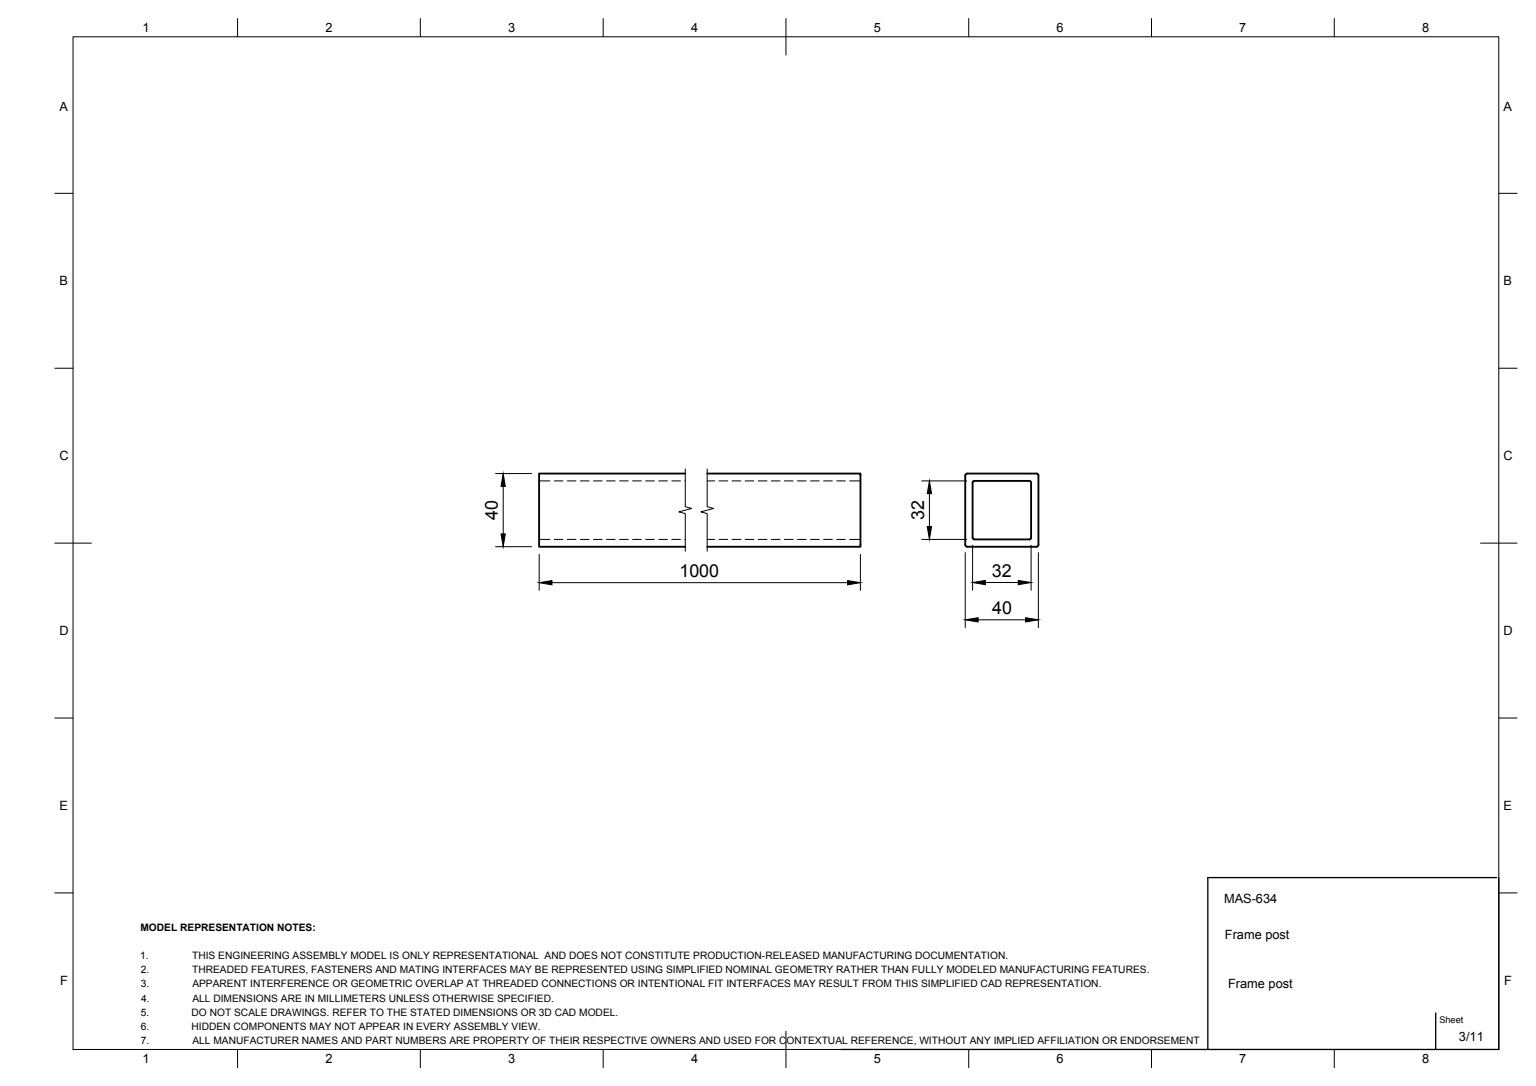
ISO-10303-21;
HEADER;
/* Generated by software containing ST-Developer
 * from STEP Tools, Inc. (www.steptools.com) 
 */

FILE_DESCRIPTION(
/* description */ ('Independent AHU equipment rack. Nominal800x600 frame on1000long40squa
re aluminum posts; two removable notched shelves; welded perimeter/cro
ss rails and rear gussets; two mounting channels; four isolation pads 
and anchor-ready feet. Imported native extrusion library retained and 
cut-length parameters customized per family. Shelf hardware uses model
ed M6 rivet nuts and screws. Weld design, floor anchors and load ratin
g require engineering selection.'),
/* implementation_level */ '2;1');

FILE_NAME(
/* name */ 'Frame post.step',
/* time_stamp */ '2026-11-07T19:04:45-08:00',
/* author */ (''),
/* organization */ (''),
/* preprocessor_version */ 'ST-DEVELOPER v20.2',
/* originating_system */ 'Autodesk Translation Framework v15.17.0.0',
/* authorisation */ '');

FILE_SCHEMA (('AUTOMOTIVE_DESIGN { 1 0 10303 214 3 1 1 }'));
ENDSEC;

DATA;
#10=MECHANICAL_DESIGN_GEOMETRIC_PRESENTATION_REPRESENTATION('',(#335),#9777);
#313=SHAPE_REPRESENTATION_RELATIONSHIP('SRR','None',#9857,#324);
#324=ADVANCED_BREP_SHAPE_REPRESENTATION('',(#346),#9766);
#335=STYLED_ITEM('',(#9921),#346);
#346=MANIFOLD_SOLID_BREP('Aluminum square hollow profile',#3840);
#357=FACE_BOUND('',#703,.T.);
#358=FACE_BOUND('',#719,.T.);
#410=PLANE('',#3978);
#411=PLANE('',#3979);
#412=PLANE('',#3989);
#413=PLANE('',#3996);
#414=PLANE('',#3999);
#415=PLANE('',#4002);
#416=PLANE('',#4005);
#417=PLANE('',#4006);
#418=PLANE('',#4007);
#419=PLANE('',#4008);
#502=FACE_OUTER_BOUND('',#700,.T.);
#503=FACE_OUTER_BOUND('',#701,.T.);
#504=FACE_OUTER_BOUND('',#702,.T.);
#505=FACE_OUTER_BOUND('',#704,.T.);
#506=FACE_OUTER_BOUND('',#705,.T.);
#507=FACE_OUTER_BOUND('',#706,.T.);
#508=FACE_OUTER_BOUND('',#707,.T.);
#509=FACE_OUTER_BOUND('',#708,.T.);
#510=FACE_OUTER_BOUND('',#709,.T.);
#511=FACE_OUTER_BOUND('',#710,.T.);
#512=FACE_OUTER_BOUND('',#711,.T.);
#513=FACE_OUTER_BOUND('',#712,.T.);
#514=FACE_OUTER_BOUND('',#713,.T.);
#515=FACE_OUTER_BOUND('',#714,.T.);
#516=FACE_OUTER_BOUND('',#715,.T.);
#517=FACE_OUTER_BOUND('',#716,.T.);
#518=FACE_OUTER_BOUND('',#717,.T.);
#519=FACE_OUTER_BOUND('',#718,.T.);
#700=EDGE_LOOP('',(#2515,#2516,#2517,#2518));
#701=EDGE_LOOP('',(#2519,#2520,#2521,#2522));
#702=EDGE_LOOP('',(#2523,#2524,#2525,#2526,#2527,#2528,#2529,#2530));
#703=EDGE_LOOP('',(#2531,#2532,#2533,#2534,#2535,#2536,#2537,#2538));
#704=EDGE_LOOP('',(#2539,#2540,#2541,#2542));
#705=EDGE_LOOP('',(#2543,#2544,#2545,#2546));
#706=EDGE_LOOP('',(#2547,#2548,#2549,#2550));
#707=EDGE_LOOP('',(#2551,#2552,#2553,#2554));
#708=EDGE_LOOP('',(#2555,#2556,#2557,#2558));
#709=EDGE_LOOP('',(#2559,#2560,#2561,#2562));
#710=EDGE_LOOP('',(#2563,#2564,#2565,#2566));
#711=EDGE_LOOP('',(#2567,#2568,#2569,#2570));
#712=EDGE_LOOP('',(#2571,#2572,#2573,#2574));
#713=EDGE_LOOP('',(#2575,#2576,#2577,#2578));
#714=EDGE_LOOP('',(#2579,#2580,#2581,#2582));
#715=EDGE_LOOP('',(#2583,#2584,#2585,#2586));
#716=EDGE_LOOP('',(#2587,#2588,#2589,#2590));
#717=EDGE_LOOP('',(#2591,#2592,#2593,#2594));
#718=EDGE_LOOP('',(#2595,#2596,#2597,#2598,#2599,#2600,#2601,#2602));
#719=EDGE_LOOP('',(#2603,#2604,#2605,#2606,#2607,#2608,#2609,#2610));
#951=LINE('',#5410,#1244);
#952=LINE('',#5413,#1245);
#953=LINE('',#5416,#1246);
#954=LINE('',#5418,#1247);
#955=LINE('',#5419,#1248);
#956=LINE('',#5422,#1249);
#957=LINE('',#5426,#1250);
#958=LINE('',#5430,#1251);
#959=LINE('',#5434,#1252);
#960=LINE('',#5438,#1253);
#961=LINE('',#5442,#1254);
#962=LINE('',#5446,#1255);
#963=LINE('',#5450,#1256);
#964=LINE('',#5453,#1257);
#965=LINE('',#5456,#1258);
#966=LINE('',#5457,#1259);
#967=LINE('',#5461,#1260);
#968=LINE('',#5464,#1261);
#969=LINE('',#5470,#1262);
#970=LINE('',#5471,#1263);
#971=LINE('',#5474,#1264);
#972=LINE('',#5475,#1265);
#973=LINE('',#5479,#1266);
#974=LINE('',#5482,#1267);
#975=LINE('',#5483,#1268);
#976=LINE('',#5487,#1269);
#977=LINE('',#5490,#1270);
#978=LINE('',#5491,#1271);
#979=LINE('',#5495,#1272);
#980=LINE('',#5497,#1273);
#981=LINE('',#5499,#1274);
#982=LINE('',#5501,#1275);
#1244=VECTOR('',#4360,10.);
#1245=VECTOR('',#4363,10.);
#1246=VECTOR('',#4366,10.);
#1247=VECTOR('',#4367,10.);
#1248=VECTOR('',#4368,10.);
#1249=VECTOR('',#4371,10.);
#1250=VECTOR('',#4374,10.);
#1251=VECTOR('',#4377,10.);
#1252=VECTOR('',#4380,10.);
#1253=VECTOR('',#4383,10.);
#1254=VECTOR('',#4386,10.);
#1255=VECTOR('',#4389,10.);
#1256=VECTOR('',#4394,10.);
#1257=VECTOR('',#4397,10.);
#1258=VECTOR('',#4400,10.);
#1259=VECTOR('',#4401,10.);
#1260=VECTOR('',#4406,10.);
#1261=VECTOR('',#4409,10.);
#1262=VECTOR('',#4416,10.);
#1263=VECTOR('',#4417,10.);
#1264=VECTOR('',#4420,10.);
#1265=VECTOR('',#4421,10.);
#1266=VECTOR('',#4426,10.);
#1267=VECTOR('',#4429,10.);
#1268=VECTOR('',#4430,10.);
#1269=VECTOR('',#4435,10.);
#1270=VECTOR('',#4438,10.);
#1271=VECTOR('',#4439,10.);
#1272=VECTOR('',#4444,10.);
#1273=VECTOR('',#4447,10.);
#1274=VECTOR('',#4450,10.);
#1275=VECTOR('',#4453,10.);
#1537=CIRCLE('',#3976,1.);
#1538=CIRCLE('',#3977,1.);
#1539=CIRCLE('',#3980,1.);
#1540=CIRCLE('',#3981,1.);
#1541=CIRCLE('',#3982,1.);
#1542=CIRCLE('',#3983,1.);
#1543=CIRCLE('',#3984,1.);
#1544=CIRCLE('',#3985,1.);
#1545=CIRCLE('',#3986,1.);
#1546=CIRCLE('',#3988,1.);
#1547=CIRCLE('',#3991,1.);
#1548=CIRCLE('',#3993,1.);
#1549=CIRCLE('',#3995,1.);
#1550=CIRCLE('',#3998,1.);
#1551=CIRCLE('',#4001,1.);
#1552=CIRCLE('',#4004,1.);
#1660=VERTEX_POINT('',#5406);
#1661=VERTEX_POINT('',#5407);
#1662=VERTEX_POINT('',#5409);
#1663=VERTEX_POINT('',#5411);
#1664=VERTEX_POINT('',#5415);
#1665=VERTEX_POINT('',#5417);
#1666=VERTEX_POINT('',#5421);
#1667=VERTEX_POINT('',#5423);
#1668=VERTEX_POINT('',#5425);
#1669=VERTEX_POINT('',#5427);
#1670=VERTEX_POINT('',#5429);
#1671=VERTEX_POINT('',#5432);
#1672=VERTEX_POINT('',#5433);
#1673=VERTEX_POINT('',#5435);
#1674=VERTEX_POINT('',#5437);
#1675=VERTEX_POINT('',#5439);
#1676=VERTEX_POINT('',#5441);
#1677=VERTEX_POINT('',#5443);
#1678=VERTEX_POINT('',#5445);
#1679=VERTEX_POINT('',#5449);
#1680=VERTEX_POINT('',#5451);
#1681=VERTEX_POINT('',#5455);
#1682=VERTEX_POINT('',#5459);
#1683=VERTEX_POINT('',#5463);
#1684=VERTEX_POINT('',#5467);
#1685=VERTEX_POINT('',#5468);
#1686=VERTEX_POINT('',#5473);
#1687=VERTEX_POINT('',#5477);
#1688=VERTEX_POINT('',#5481);
#1689=VERTEX_POINT('',#5485);
#1690=VERTEX_POINT('',#5489);
#1691=VERTEX_POINT('',#5493);
#2002=EDGE_CURVE('',#1660,#1661,#1537,.T.);
#2003=EDGE_CURVE('',#1661,#1662,#951,.T.);
#2004=EDGE_CURVE('',#1662,#1663,#1538,.T.);
#2005=EDGE_CURVE('',#1663,#1660,#952,.T.);
#2006=EDGE_CURVE('',#1664,#1661,#953,.T.);
#2007=EDGE_CURVE('',#1665,#1664,#954,.T.);
#2008=EDGE_CURVE('',#1665,#1662,#955,.T.);
#2009=EDGE_CURVE('',#1660,#1666,#956,.T.);
#2010=EDGE_CURVE('',#1667,#1666,#1539,.T.);
#2011=EDGE_CURVE('',#1667,#1668,#957,.T.);
#2012=EDGE_CURVE('',#1669,#1668,#1540,.T.);
#2013=EDGE_CURVE('',#1669,#1670,#958,.T.);
#2014=EDGE_CURVE('',#1664,#1670,#1541,.T.);
#2015=EDGE_CURVE('',#1671,#1672,#959,.T.);
#2016=EDGE_CURVE('',#1673,#1672,#1542,.T.);
#2017=EDGE_CURVE('',#1673,#1674,#960,.T.);
#2018=EDGE_CURVE('',#1675,#1674,#1543,.T.);
#2019=EDGE_CURVE('',#1675,#1676,#961,.T.);
#2020=EDGE_CURVE('',#1677,#1676,#1544,.T.);
#2021=EDGE_CURVE('',#1677,#1678,#962,.T.);
#2022=EDGE_CURVE('',#1671,#1678,#1545,.T.);
#2023=EDGE_CURVE('',#1666,#1679,#963,.T.);
#2024=EDGE_CURVE('',#1679,#1680,#1546,.T.);
#2025=EDGE_CURVE('',#1680,#1667,#964,.T.);
#2026=EDGE_CURVE('',#1680,#1681,#965,.T.);
#2027=EDGE_CURVE('',#1668,#1681,#966,.T.);
#2028=EDGE_CURVE('',#1681,#1682,#1547,.T.);
#2029=EDGE_CURVE('',#1682,#1669,#967,.T.);
#2030=EDGE_CURVE('',#1670,#1683,#968,.T.);
#2031=EDGE_CURVE('',#1683,#1665,#1548,.T.);
#2032=EDGE_CURVE('',#1684,#1685,#1549,.T.);
#2033=EDGE_CURVE('',#1685,#1673,#969,.T.);
#2034=EDGE_CURVE('',#1672,#1684,#970,.T.);
#2035=EDGE_CURVE('',#1685,#1686,#971,.T.);
#2036=EDGE_CURVE('',#1674,#1686,#972,.T.);
#2037=EDGE_CURVE('',#1686,#1687,#1550,.T.);
#2038=EDGE_CURVE('',#1687,#1675,#973,.T.);
#2039=EDGE_CURVE('',#1687,#1688,#974,.T.);
#2040=EDGE_CURVE('',#1676,#1688,#975,.T.);
#2041=EDGE_CURVE('',#1688,#1689,#1551,.T.);
#2042=EDGE_CURVE('',#1689,#1677,#976,.T.);
#2043=EDGE_CURVE('',#1689,#1690,#977,.T.);
#2044=EDGE_CURVE('',#1678,#1690,#978,.T.);
#2045=EDGE_CURVE('',#1690,#1691,#1552,.T.);
#2046=EDGE_CURVE('',#1691,#1671,#979,.T.);
#2047=EDGE_CURVE('',#1691,#1684,#980,.T.);
#2048=EDGE_CURVE('',#1682,#1683,#981,.T.);
#2049=EDGE_CURVE('',#1663,#1679,#982,.T.);
#2515=ORIENTED_EDGE('',*,*,#2002,.T.);
#2516=ORIENTED_EDGE('',*,*,#2003,.T.);
#2517=ORIENTED_EDGE('',*,*,#2004,.T.);
#2518=ORIENTED_EDGE('',*,*,#2005,.T.);
#2519=ORIENTED_EDGE('',*,*,#2003,.F.);
#2520=ORIENTED_EDGE('',*,*,#2006,.F.);
#2521=ORIENTED_EDGE('',*,*,#2007,.F.);
#2522=ORIENTED_EDGE('',*,*,#2008,.T.);
#2523=ORIENTED_EDGE('',*,*,#2002,.F.);
#2524=ORIENTED_EDGE('',*,*,#2009,.T.);
#2525=ORIENTED_EDGE('',*,*,#2010,.F.);
#2526=ORIENTED_EDGE('',*,*,#2011,.T.);
#2527=ORIENTED_EDGE('',*,*,#2012,.F.);
#2528=ORIENTED_EDGE('',*,*,#2013,.T.);
#2529=ORIENTED_EDGE('',*,*,#2014,.F.);
#2530=ORIENTED_EDGE('',*,*,#2006,.T.);
#2531=ORIENTED_EDGE('',*,*,#2015,.T.);
#2532=ORIENTED_EDGE('',*,*,#2016,.F.);
#2533=ORIENTED_EDGE('',*,*,#2017,.T.);
#2534=ORIENTED_EDGE('',*,*,#2018,.F.);
#2535=ORIENTED_EDGE('',*,*,#2019,.T.);
#2536=ORIENTED_EDGE('',*,*,#2020,.F.);
#2537=ORIENTED_EDGE('',*,*,#2021,.T.);
#2538=ORIENTED_EDGE('',*,*,#2022,.F.);
#2539=ORIENTED_EDGE('',*,*,#2010,.T.);
#2540=ORIENTED_EDGE('',*,*,#2023,.T.);
#2541=ORIENTED_EDGE('',*,*,#2024,.T.);
#2542=ORIENTED_EDGE('',*,*,#2025,.T.);
#2543=ORIENTED_EDGE('',*,*,#2025,.F.);
#2544=ORIENTED_EDGE('',*,*,#2026,.T.);
#2545=ORIENTED_EDGE('',*,*,#2027,.F.);
#2546=ORIENTED_EDGE('',*,*,#2011,.F.);
#2547=ORIENTED_EDGE('',*,*,#2012,.T.);
#2548=ORIENTED_EDGE('',*,*,#2027,.T.);
#2549=ORIENTED_EDGE('',*,*,#2028,.T.);
#2550=ORIENTED_EDGE('',*,*,#2029,.T.);
#2551=ORIENTED_EDGE('',*,*,#2014,.T.);
#2552=ORIENTED_EDGE('',*,*,#2030,.T.);
#2553=ORIENTED_EDGE('',*,*,#2031,.T.);
#2554=ORIENTED_EDGE('',*,*,#2007,.T.);
#2555=ORIENTED_EDGE('',*,*,#2032,.T.);
#2556=ORIENTED_EDGE('',*,*,#2033,.T.);
#2557=ORIENTED_EDGE('',*,*,#2016,.T.);
#2558=ORIENTED_EDGE('',*,*,#2034,.T.);
#2559=ORIENTED_EDGE('',*,*,#2033,.F.);
#2560=ORIENTED_EDGE('',*,*,#2035,.T.);
#2561=ORIENTED_EDGE('',*,*,#2036,.F.);
#2562=ORIENTED_EDGE('',*,*,#2017,.F.);
#2563=ORIENTED_EDGE('',*,*,#2037,.T.);
#2564=ORIENTED_EDGE('',*,*,#2038,.T.);
#2565=ORIENTED_EDGE('',*,*,#2018,.T.);
#2566=ORIENTED_EDGE('',*,*,#2036,.T.);
#2567=ORIENTED_EDGE('',*,*,#2038,.F.);
#2568=ORIENTED_EDGE('',*,*,#2039,.T.);
#2569=ORIENTED_EDGE('',*,*,#2040,.F.);
#2570=ORIENTED_EDGE('',*,*,#2019,.F.);
#2571=ORIENTED_EDGE('',*,*,#2041,.T.);
#2572=ORIENTED_EDGE('',*,*,#2042,.T.);
#2573=ORIENTED_EDGE('',*,*,#2020,.T.);
#2574=ORIENTED_EDGE('',*,*,#2040,.T.);
#2575=ORIENTED_EDGE('',*,*,#2042,.F.);
#2576=ORIENTED_EDGE('',*,*,#2043,.T.);
#2577=ORIENTED_EDGE('',*,*,#2044,.F.);
#2578=ORIENTED_EDGE('',*,*,#2021,.F.);
#2579=ORIENTED_EDGE('',*,*,#2045,.T.);
#2580=ORIENTED_EDGE('',*,*,#2046,.T.);
#2581=ORIENTED_EDGE('',*,*,#2022,.T.);
#2582=ORIENTED_EDGE('',*,*,#2044,.T.);
#2583=ORIENTED_EDGE('',*,*,#2034,.F.);
#2584=ORIENTED_EDGE('',*,*,#2015,.F.);
#2585=ORIENTED_EDGE('',*,*,#2046,.F.);
#2586=ORIENTED_EDGE('',*,*,#2047,.T.);
#2587=ORIENTED_EDGE('',*,*,#2029,.F.);
#2588=ORIENTED_EDGE('',*,*,#2048,.T.);
#2589=ORIENTED_EDGE('',*,*,#2030,.F.);
#2590=ORIENTED_EDGE('',*,*,#2013,.F.);
#2591=ORIENTED_EDGE('',*,*,#2005,.F.);
#2592=ORIENTED_EDGE('',*,*,#2049,.T.);
#2593=ORIENTED_EDGE('',*,*,#2023,.F.);
#2594=ORIENTED_EDGE('',*,*,#2009,.F.);
#2595=ORIENTED_EDGE('',*,*,#2004,.F.);
#2596=ORIENTED_EDGE('',*,*,#2008,.F.);
#2597=ORIENTED_EDGE('',*,*,#2031,.F.);
#2598=ORIENTED_EDGE('',*,*,#2048,.F.);
#2599=ORIENTED_EDGE('',*,*,#2028,.F.);
#2600=ORIENTED_EDGE('',*,*,#2026,.F.);
#2601=ORIENTED_EDGE('',*,*,#2024,.F.);
#2602=ORIENTED_EDGE('',*,*,#2049,.F.);
#2603=ORIENTED_EDGE('',*,*,#2045,.F.);
#2604=ORIENTED_EDGE('',*,*,#2043,.F.);
#2605=ORIENTED_EDGE('',*,*,#2041,.F.);
#2606=ORIENTED_EDGE('',*,*,#2039,.F.);
#2607=ORIENTED_EDGE('',*,*,#2037,.F.);
#2608=ORIENTED_EDGE('',*,*,#2035,.F.);
#2609=ORIENTED_EDGE('',*,*,#2032,.F.);
#2610=ORIENTED_EDGE('',*,*,#2047,.F.);
#3541=CYLINDRICAL_SURFACE('',#3975,1.);
#3542=CYLINDRICAL_SURFACE('',#3987,1.);
#3543=CYLINDRICAL_SURFACE('',#3990,1.);
#3544=CYLINDRICAL_SURFACE('',#3992,1.);
#3545=CYLINDRICAL_SURFACE('',#3994,1.);
#3546=CYLINDRICAL_SURFACE('',#3997,1.);
#3547=CYLINDRICAL_SURFACE('',#4000,1.);
#3548=CYLINDRICAL_SURFACE('',#4003,1.);
#3642=ADVANCED_FACE('',(#502),#3541,.T.);
#3643=ADVANCED_FACE('',(#503),#410,.T.);
#3644=ADVANCED_FACE('',(#504,#357),#411,.T.);
#3645=ADVANCED_FACE('',(#505),#3542,.T.);
#3646=ADVANCED_FACE('',(#506),#412,.T.);
#3647=ADVANCED_FACE('',(#507),#3543,.T.);
#3648=ADVANCED_FACE('',(#508),#3544,.T.);
#3649=ADVANCED_FACE('',(#509),#3545,.F.);
#3650=ADVANCED_FACE('',(#510),#413,.T.);
#3651=ADVANCED_FACE('',(#511),#3546,.F.);
#3652=ADVANCED_FACE('',(#512),#414,.T.);
#3653=ADVANCED_FACE('',(#513),#3547,.F.);
#3654=ADVANCED_FACE('',(#514),#415,.T.);
#3655=ADVANCED_FACE('',(#515),#3548,.F.);
#3656=ADVANCED_FACE('',(#516),#416,.T.);
#3657=ADVANCED_FACE('',(#517),#417,.T.);
#3658=ADVANCED_FACE('',(#518),#418,.T.);
#3659=ADVANCED_FACE('',(#519,#358),#419,.F.);
#3840=CLOSED_SHELL('',(#3642,#3643,#3644,#3645,#3646,#3647,#3648,#3649,
#3650,#3651,#3652,#3653,#3654,#3655,#3656,#3657,#3658,#3659));
#3974=AXIS2_PLACEMENT_3D('',#5404,#4354,#4355);
#3975=AXIS2_PLACEMENT_3D('',#5405,#4356,#4357);
#3976=AXIS2_PLACEMENT_3D('',#5408,#4358,#4359);
#3977=AXIS2_PLACEMENT_3D('',#5412,#4361,#4362);
#3978=AXIS2_PLACEMENT_3D('',#5414,#4364,#4365);
#3979=AXIS2_PLACEMENT_3D('',#5420,#4369,#4370);
#3980=AXIS2_PLACEMENT_3D('',#5424,#4372,#4373);
#3981=AXIS2_PLACEMENT_3D('',#5428,#4375,#4376);
#3982=AXIS2_PLACEMENT_3D('',#5431,#4378,#4379);
#3983=AXIS2_PLACEMENT_3D('',#5436,#4381,#4382);
#3984=AXIS2_PLACEMENT_3D('',#5440,#4384,#4385);
#3985=AXIS2_PLACEMENT_3D('',#5444,#4387,#4388);
#3986=AXIS2_PLACEMENT_3D('',#5447,#4390,#4391);
#3987=AXIS2_PLACEMENT_3D('',#5448,#4392,#4393);
#3988=AXIS2_PLACEMENT_3D('',#5452,#4395,#4396);
#3989=AXIS2_PLACEMENT_3D('',#5454,#4398,#4399);
#3990=AXIS2_PLACEMENT_3D('',#5458,#4402,#4403);
#3991=AXIS2_PLACEMENT_3D('',#5460,#4404,#4405);
#3992=AXIS2_PLACEMENT_3D('',#5462,#4407,#4408);
#3993=AXIS2_PLACEMENT_3D('',#5465,#4410,#4411);
#3994=AXIS2_PLACEMENT_3D('',#5466,#4412,#4413);
#3995=AXIS2_PLACEMENT_3D('',#5469,#4414,#4415);
#3996=AXIS2_PLACEMENT_3D('',#5472,#4418,#4419);
#3997=AXIS2_PLACEMENT_3D('',#5476,#4422,#4423);
#3998=AXIS2_PLACEMENT_3D('',#5478,#4424,#4425);
#3999=AXIS2_PLACEMENT_3D('',#5480,#4427,#4428);
#4000=AXIS2_PLACEMENT_3D('',#5484,#4431,#4432);
#4001=AXIS2_PLACEMENT_3D('',#5486,#4433,#4434);
#4002=AXIS2_PLACEMENT_3D('',#5488,#4436,#4437);
#4003=AXIS2_PLACEMENT_3D('',#5492,#4440,#4441);
#4004=AXIS2_PLACEMENT_3D('',#5494,#4442,#4443);
#4005=AXIS2_PLACEMENT_3D('',#5496,#4445,#4446);
#4006=AXIS2_PLACEMENT_3D('',#5498,#4448,#4449);
#4007=AXIS2_PLACEMENT_3D('',#5500,#4451,#4452);
#4008=AXIS2_PLACEMENT_3D('',#5502,#4454,#4455);
#4354=DIRECTION('axis',(0.,0.,1.));
#4355=DIRECTION('refdir',(1.,0.,0.));
#4356=DIRECTION('center_axis',(0.,0.,1.));
#4357=DIRECTION('ref_axis',(-0.707106781186548,-0.707106781186548,0.));
#4358=DIRECTION('center_axis',(0.,0.,-1.));
#4359=DIRECTION('ref_axis',(-0.707106781186548,-0.707106781186548,0.));
#4360=DIRECTION('',(0.,0.,-1.));
#4361=DIRECTION('center_axis',(0.,0.,1.));
#4362=DIRECTION('ref_axis',(-0.707106781186548,-0.707106781186548,0.));
#4363=DIRECTION('',(0.,0.,1.));
#4364=DIRECTION('center_axis',(-1.,0.,0.));
#4365=DIRECTION('ref_axis',(0.,-1.,0.));
#4366=DIRECTION('',(0.,-1.,0.));
#4367=DIRECTION('',(0.,0.,1.));
#4368=DIRECTION('',(0.,-1.,0.));
#4369=DIRECTION('center_axis',(0.,0.,1.));
#4370=DIRECTION('ref_axis',(1.,0.,0.));
#4371=DIRECTION('',(1.,0.,0.));
#4372=DIRECTION('center_axis',(0.,0.,-1.));
#4373=DIRECTION('ref_axis',(0.707106781186548,-0.707106781186548,0.));
#4374=DIRECTION('',(0.,1.,0.));
#4375=DIRECTION('center_axis',(0.,0.,-1.));
#4376=DIRECTION('ref_axis',(0.707106781186548,0.707106781186548,0.));
#4377=DIRECTION('',(-1.,0.,0.));
#4378=DIRECTION('center_axis',(0.,0.,-1.));
#4379=DIRECTION('ref_axis',(-0.707106781186548,0.707106781186548,0.));
#4380=DIRECTION('',(0.,1.,0.));
#4381=DIRECTION('center_axis',(0.,0.,1.));
#4382=DIRECTION('ref_axis',(-0.707106781186548,0.707106781186548,0.));
#4383=DIRECTION('',(1.,0.,0.));
#4384=DIRECTION('center_axis',(0.,0.,1.));
#4385=DIRECTION('ref_axis',(0.707106781186548,0.707106781186548,0.));
#4386=DIRECTION('',(0.,-1.,0.));
#4387=DIRECTION('center_axis',(0.,0.,1.));
#4388=DIRECTION('ref_axis',(0.707106781186548,-0.707106781186548,0.));
#4389=DIRECTION('',(-1.,0.,0.));
#4390=DIRECTION('center_axis',(0.,0.,1.));
#4391=DIRECTION('ref_axis',(-0.707106781186548,-0.707106781186548,0.));
#4392=DIRECTION('center_axis',(0.,0.,1.));
#4393=DIRECTION('ref_axis',(0.707106781186548,-0.707106781186548,0.));
#4394=DIRECTION('',(0.,0.,-1.));
#4395=DIRECTION('center_axis',(0.,0.,1.));
#4396=DIRECTION('ref_axis',(0.707106781186548,-0.707106781186548,0.));
#4397=DIRECTION('',(0.,0.,1.));
#4398=DIRECTION('center_axis',(1.,0.,0.));
#4399=DIRECTION('ref_axis',(0.,1.,0.));
#4400=DIRECTION('',(0.,1.,0.));
#4401=DIRECTION('',(0.,0.,-1.));
#4402=DIRECTION('center_axis',(0.,0.,1.));
#4403=DIRECTION('ref_axis',(0.707106781186548,0.707106781186548,0.));
#4404=DIRECTION('center_axis',(0.,0.,1.));
#4405=DIRECTION('ref_axis',(0.707106781186548,0.707106781186548,0.));
#4406=DIRECTION('',(0.,0.,1.));
#4407=DIRECTION('center_axis',(0.,0.,1.));
#4408=DIRECTION('ref_axis',(-0.707106781186548,0.707106781186548,0.));
#4409=DIRECTION('',(0.,0.,-1.));
#4410=DIRECTION('center_axis',(0.,0.,1.));
#4411=DIRECTION('ref_axis',(-0.707106781186548,0.707106781186548,0.));
#4412=DIRECTION('center_axis',(0.,0.,1.));
#4413=DIRECTION('ref_axis',(-0.707106781186548,0.707106781186548,0.));
#4414=DIRECTION('center_axis',(0.,0.,-1.));
#4415=DIRECTION('ref_axis',(-0.707106781186548,0.707106781186548,0.));
#4416=DIRECTION('',(0.,0.,1.));
#4417=DIRECTION('',(0.,0.,-1.));
#4418=DIRECTION('center_axis',(0.,-1.,0.));
#4419=DIRECTION('ref_axis',(1.,0.,0.));
#4420=DIRECTION('',(1.,0.,0.));
#4421=DIRECTION('',(0.,0.,-1.));
#4422=DIRECTION('center_axis',(0.,0.,1.));
#4423=DIRECTION('ref_axis',(0.707106781186548,0.707106781186548,0.));
#4424=DIRECTION('center_axis',(0.,0.,-1.));
#4425=DIRECTION('ref_axis',(0.707106781186548,0.707106781186548,0.));
#4426=DIRECTION('',(0.,0.,1.));
#4427=DIRECTION('center_axis',(-1.,0.,0.));
#4428=DIRECTION('ref_axis',(0.,-1.,0.));
#4429=DIRECTION('',(0.,-1.,0.));
#4430=DIRECTION('',(0.,0.,-1.));
#4431=DIRECTION('center_axis',(0.,0.,1.));
#4432=DIRECTION('ref_axis',(0.707106781186548,-0.707106781186548,0.));
#4433=DIRECTION('center_axis',(0.,0.,-1.));
#4434=DIRECTION('ref_axis',(0.707106781186548,-0.707106781186548,0.));
#4435=DIRECTION('',(0.,0.,1.));
#4436=DIRECTION('center_axis',(0.,1.,0.));
#4437=DIRECTION('ref_axis',(-1.,0.,0.));
#4438=DIRECTION('',(-1.,0.,0.));
#4439=DIRECTION('',(0.,0.,-1.));
#4440=DIRECTION('center_axis',(0.,0.,1.));
#4441=DIRECTION('ref_axis',(-0.707106781186548,-0.707106781186548,0.));
#4442=DIRECTION('center_axis',(0.,0.,-1.));
#4443=DIRECTION('ref_axis',(-0.707106781186548,-0.707106781186548,0.));
#4444=DIRECTION('',(0.,0.,1.));
#4445=DIRECTION('center_axis',(1.,0.,0.));
#4446=DIRECTION('ref_axis',(0.,1.,0.));
#4447=DIRECTION('',(0.,1.,0.));
#4448=DIRECTION('center_axis',(0.,1.,0.));
#4449=DIRECTION('ref_axis',(-1.,0.,0.));
#4450=DIRECTION('',(-1.,0.,0.));
#4451=DIRECTION('center_axis',(0.,-1.,0.));
#4452=DIRECTION('ref_axis',(1.,0.,0.));
#4453=DIRECTION('',(1.,0.,0.));
#4454=DIRECTION('center_axis',(0.,0.,1.));
#4455=DIRECTION('ref_axis',(1.,0.,0.));
#5404=CARTESIAN_POINT('',(0.,0.,0.));
#5405=CARTESIAN_POINT('Origin',(-19.,-19.,0.));
#5406=CARTESIAN_POINT('',(-19.,-20.,1000.));
#5407=CARTESIAN_POINT('',(-20.,-19.,1000.));
#5408=CARTESIAN_POINT('Origin',(-19.,-19.,1000.));
#5409=CARTESIAN_POINT('',(-20.,-19.,0.));
#5410=CARTESIAN_POINT('',(-20.,-19.,0.));
#5411=CARTESIAN_POINT('',(-19.,-20.,0.));
#5412=CARTESIAN_POINT('Origin',(-19.,-19.,0.));
#5413=CARTESIAN_POINT('',(-19.,-20.,0.));
#5414=CARTESIAN_POINT('Origin',(-20.,20.,0.));
#5415=CARTESIAN_POINT('',(-20.,19.,1000.));
#5416=CARTESIAN_POINT('',(-20.,20.,1000.));
#5417=CARTESIAN_POINT('',(-20.,19.,0.));
#5418=CARTESIAN_POINT('',(-20.,19.,0.));
#5419=CARTESIAN_POINT('',(-20.,20.,0.));
#5420=CARTESIAN_POINT('Origin',(0.,0.,1000.));
#5421=CARTESIAN_POINT('',(19.,-20.,1000.));
#5422=CARTESIAN_POINT('',(-20.,-20.,1000.));
#5423=CARTESIAN_POINT('',(20.,-19.,1000.));
#5424=CARTESIAN_POINT('Origin',(19.,-19.,1000.));
#5425=CARTESIAN_POINT('',(20.,19.,1000.));
#5426=CARTESIAN_POINT('',(20.,-20.,1000.));
#5427=CARTESIAN_POINT('',(19.,20.,1000.));
#5428=CARTESIAN_POINT('Origin',(19.,19.,1000.));
#5429=CARTESIAN_POINT('',(-19.,20.,1000.));
#5430=CARTESIAN_POINT('',(20.,20.,1000.));
#5431=CARTESIAN_POINT('Origin',(-19.,19.,1000.));
#5432=CARTESIAN_POINT('',(-16.,-15.,1000.));
#5433=CARTESIAN_POINT('',(-16.,15.,1000.));
#5434=CARTESIAN_POINT('',(-16.,16.,1000.));
#5435=CARTESIAN_POINT('',(-15.,16.,1000.));
#5436=CARTESIAN_POINT('Origin',(-15.,15.,1000.));
#5437=CARTESIAN_POINT('',(15.,16.,1000.));
#5438=CARTESIAN_POINT('',(16.,16.,1000.));
#5439=CARTESIAN_POINT('',(16.,15.,1000.));
#5440=CARTESIAN_POINT('Origin',(15.,15.,1000.));
#5441=CARTESIAN_POINT('',(16.,-15.,1000.));
#5442=CARTESIAN_POINT('',(16.,-16.,1000.));
#5443=CARTESIAN_POINT('',(15.,-16.,1000.));
#5444=CARTESIAN_POINT('Origin',(15.,-15.,1000.));
#5445=CARTESIAN_POINT('',(-15.,-16.,1000.));
#5446=CARTESIAN_POINT('',(-16.,-16.,1000.));
#5447=CARTESIAN_POINT('Origin',(-15.,-15.,1000.));
#5448=CARTESIAN_POINT('Origin',(19.,-19.,0.));
#5449=CARTESIAN_POINT('',(19.,-20.,0.));
#5450=CARTESIAN_POINT('',(19.,-20.,0.));
#5451=CARTESIAN_POINT('',(20.,-19.,0.));
#5452=CARTESIAN_POINT('Origin',(19.,-19.,0.));
#5453=CARTESIAN_POINT('',(20.,-19.,0.));
#5454=CARTESIAN_POINT('Origin',(20.,-20.,0.));
#5455=CARTESIAN_POINT('',(20.,19.,0.));
#5456=CARTESIAN_POINT('',(20.,-20.,0.));
#5457=CARTESIAN_POINT('',(20.,19.,0.));
#5458=CARTESIAN_POINT('Origin',(19.,19.,0.));
#5459=CARTESIAN_POINT('',(19.,20.,0.));
#5460=CARTESIAN_POINT('Origin',(19.,19.,0.));
#5461=CARTESIAN_POINT('',(19.,20.,0.));
#5462=CARTESIAN_POINT('Origin',(-19.,19.,0.));
#5463=CARTESIAN_POINT('',(-19.,20.,0.));
#5464=CARTESIAN_POINT('',(-19.,20.,0.));
#5465=CARTESIAN_POINT('Origin',(-19.,19.,0.));
#5466=CARTESIAN_POINT('Origin',(-15.,15.,0.));
#5467=CARTESIAN_POINT('',(-16.,15.,0.));
#5468=CARTESIAN_POINT('',(-15.,16.,0.));
#5469=CARTESIAN_POINT('Origin',(-15.,15.,0.));
#5470=CARTESIAN_POINT('',(-15.,16.,0.));
#5471=CARTESIAN_POINT('',(-16.,15.,0.));
#5472=CARTESIAN_POINT('Origin',(-16.,16.,0.));
#5473=CARTESIAN_POINT('',(15.,16.,0.));
#5474=CARTESIAN_POINT('',(16.,16.,0.));
#5475=CARTESIAN_POINT('',(15.,16.,0.));
#5476=CARTESIAN_POINT('Origin',(15.,15.,0.));
#5477=CARTESIAN_POINT('',(16.,15.,0.));
#5478=CARTESIAN_POINT('Origin',(15.,15.,0.));
#5479=CARTESIAN_POINT('',(16.,15.,0.));
#5480=CARTESIAN_POINT('Origin',(16.,16.,0.));
#5481=CARTESIAN_POINT('',(16.,-15.,0.));
#5482=CARTESIAN_POINT('',(16.,-16.,0.));
#5483=CARTESIAN_POINT('',(16.,-15.,0.));
#5484=CARTESIAN_POINT('Origin',(15.,-15.,0.));
#5485=CARTESIAN_POINT('',(15.,-16.,0.));
#5486=CARTESIAN_POINT('Origin',(15.,-15.,0.));
#5487=CARTESIAN_POINT('',(15.,-16.,0.));
#5488=CARTESIAN_POINT('Origin',(16.,-16.,0.));
#5489=CARTESIAN_POINT('',(-15.,-16.,0.));
#5490=CARTESIAN_POINT('',(-16.,-16.,0.));
#5491=CARTESIAN_POINT('',(-15.,-16.,0.));
#5492=CARTESIAN_POINT('Origin',(-15.,-15.,0.));
#5493=CARTESIAN_POINT('',(-16.,-15.,0.));
#5494=CARTESIAN_POINT('Origin',(-15.,-15.,0.));
#5495=CARTESIAN_POINT('',(-16.,-15.,0.));
#5496=CARTESIAN_POINT('Origin',(-16.,-16.,0.));
#5497=CARTESIAN_POINT('',(-16.,16.,0.));
#5498=CARTESIAN_POINT('Origin',(20.,20.,0.));
#5499=CARTESIAN_POINT('',(20.,20.,0.));
#5500=CARTESIAN_POINT('Origin',(-20.,-20.,0.));
#5501=CARTESIAN_POINT('',(-20.,-20.,0.));
#5502=CARTESIAN_POINT('Origin',(0.,0.,0.));
#9753=UNCERTAINTY_MEASURE_WITH_UNIT(LENGTH_MEASURE(0.01),#9778,
'DISTANCE_ACCURACY_VALUE',
'Maximum model space distance between geometric entities at asserted c
onnectivities');
#9764=UNCERTAINTY_MEASURE_WITH_UNIT(LENGTH_MEASURE(0.01),#9778,
'DISTANCE_ACCURACY_VALUE',
'Maximum model space distance between geometric entities at asserted c
onnectivities');
#9766=(
GEOMETRIC_REPRESENTATION_CONTEXT(3)
GLOBAL_UNCERTAINTY_ASSIGNED_CONTEXT((#9753))
GLOBAL_UNIT_ASSIGNED_CONTEXT((#9778,#9780,#9781))
REPRESENTATION_CONTEXT('','3D')
);
#9777=(
GEOMETRIC_REPRESENTATION_CONTEXT(3)
GLOBAL_UNCERTAINTY_ASSIGNED_CONTEXT((#9764))
GLOBAL_UNIT_ASSIGNED_CONTEXT((#9778,#9780,#9781))
REPRESENTATION_CONTEXT('','3D')
);
#9778=(
LENGTH_UNIT()
NAMED_UNIT(*)
SI_UNIT(.MILLI.,.METRE.)
);
#9780=(
NAMED_UNIT(*)
PLANE_ANGLE_UNIT()
SI_UNIT($,.RADIAN.)
);
#9781=(
NAMED_UNIT(*)
SI_UNIT($,.STERADIAN.)
SOLID_ANGLE_UNIT()
);
#9783=SHAPE_DEFINITION_REPRESENTATION(#9795,#9857);
#9795=PRODUCT_DEFINITION_SHAPE('',$,#9870);
#9857=SHAPE_REPRESENTATION('',(#3974),#9766);
#9868=PRODUCT_DEFINITION_CONTEXT('part definition',#9906,'design');
#9870=PRODUCT_DEFINITION('Frame post','Frame post',#9882,#9868);
#9882=PRODUCT_DEFINITION_FORMATION('',$,#9909);
#9906=APPLICATION_CONTEXT(
'Core Data for Automotive Mechanical Design Process');
#9907=PRODUCT_CONTEXT('part definition',#9906,'mechanical');
#9909=PRODUCT('Frame post','Frame post',
'Independent aluminum extrusion section. Whole-mm nominal die dimensio
ns; parametric saw-cut length. Select structural loading, tolerances a
nd finish for the assembly application.',(#9907));
#9921=PRESENTATION_STYLE_ASSIGNMENT((#9932));
#9932=SURFACE_STYLE_USAGE(.BOTH.,#9943);
#9943=SURFACE_SIDE_STYLE('',(#9954));
#9954=SURFACE_STYLE_FILL_AREA(#9965);
#9965=FILL_AREA_STYLE('Frame gray',(#9976));
#9976=FILL_AREA_STYLE_COLOUR('Frame gray',#9987);
#9987=COLOUR_RGB('Frame gray',0.407843137254902,0.447058823529412,0.498039215686275);
ENDSEC;
END-ISO-10303-21;
